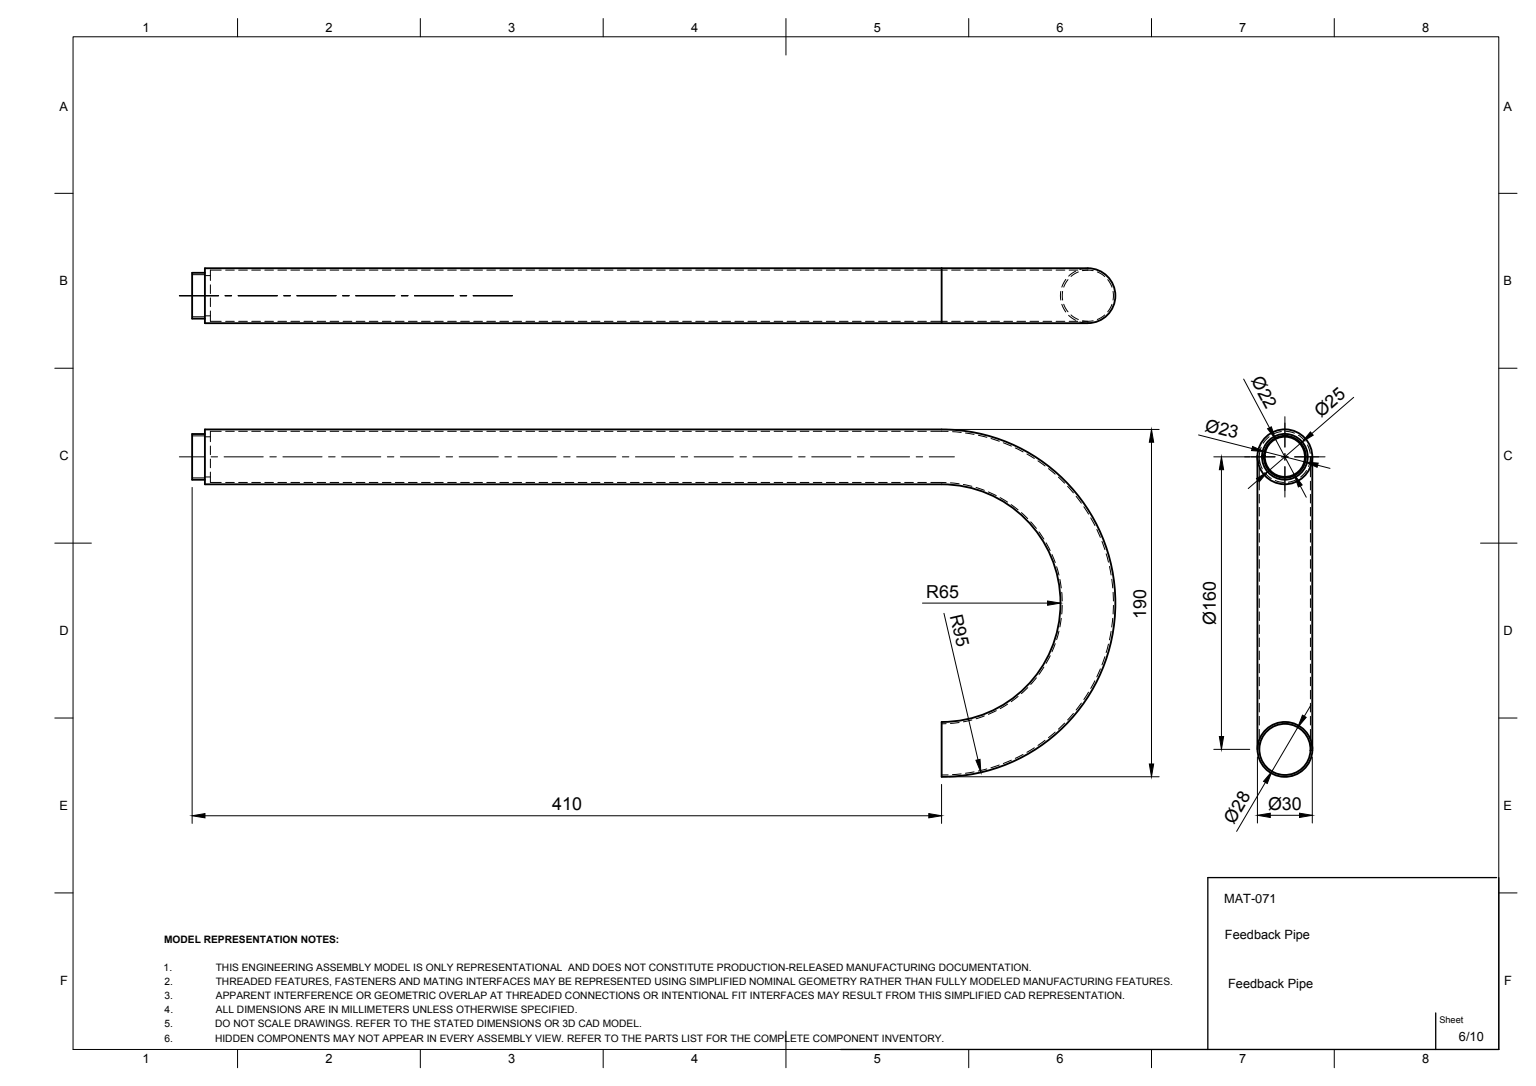
ISO-10303-21;
HEADER;
/* Generated by software containing ST-Developer
 * from STEP Tools, Inc. (www.steptools.com) 
 */

FILE_DESCRIPTION(
/* description */ (''),
/* implementation_level */ '2;1');

FILE_NAME(
/* name */ 'Feedback Pipe.step',
/* time_stamp */ '2026-10-24T12:24:47-07:00',
/* author */ (''),
/* organization */ (''),
/* preprocessor_version */ 'ST-DEVELOPER v20.2',
/* originating_system */ 'Autodesk Translation Framework v15.15.0.0',
/* authorisation */ '');

FILE_SCHEMA (('AUTOMOTIVE_DESIGN { 1 0 10303 214 3 1 1 }'));
ENDSEC;

DATA;
#10=MECHANICAL_DESIGN_GEOMETRIC_PRESENTATION_REPRESENTATION('',(#61),#13594);
#11=TOROIDAL_SURFACE('',#3227,80.0000000000001,15.);
#12=TOROIDAL_SURFACE('',#3233,80.0000000000001,14.);
#49=SHAPE_REPRESENTATION_RELATIONSHIP('SRR','None',#13629,#55);
#55=ADVANCED_BREP_SHAPE_REPRESENTATION('',(#67),#13592);
#61=STYLED_ITEM('',(#13667),#67);
#67=MANIFOLD_SOLID_BREP('Feedback Pipe',#2968);
#99=PLANE('',#3224);
#100=PLANE('',#3239);
#101=PLANE('',#3247);
#102=PLANE('',#3248);
#103=PLANE('',#3251);
#129=FACE_BOUND('',#538,.T.);
#130=FACE_BOUND('',#544,.T.);
#131=FACE_BOUND('',#548,.T.);
#132=FACE_BOUND('',#550,.T.);
#133=FACE_BOUND('',#553,.T.);
#185=CIRCLE('',#3225,15.);
#186=CIRCLE('',#3226,14.);
#187=CIRCLE('',#3228,15.);
#188=CIRCLE('',#3229,15.);
#189=CIRCLE('',#3230,65.0000000000001);
#190=CIRCLE('',#3232,15.);
#191=CIRCLE('',#3234,66.0000000000001);
#192=CIRCLE('',#3235,14.);
#193=CIRCLE('',#3236,14.);
#194=CIRCLE('',#3238,14.);
#195=CIRCLE('',#3240,11.);
#196=CIRCLE('',#3242,12.5);
#197=CIRCLE('',#3243,12.5);
#198=CIRCLE('',#3245,11.5);
#199=CIRCLE('',#3246,11.5);
#200=CIRCLE('',#3249,11.);
#350=FACE_OUTER_BOUND('',#537,.T.);
#351=FACE_OUTER_BOUND('',#539,.T.);
#352=FACE_OUTER_BOUND('',#540,.T.);
#353=FACE_OUTER_BOUND('',#541,.T.);
#354=FACE_OUTER_BOUND('',#542,.T.);
#355=FACE_OUTER_BOUND('',#543,.T.);
#356=FACE_OUTER_BOUND('',#545,.T.);
#357=FACE_OUTER_BOUND('',#546,.T.);
#358=FACE_OUTER_BOUND('',#547,.T.);
#359=FACE_OUTER_BOUND('',#549,.T.);
#360=FACE_OUTER_BOUND('',#551,.T.);
#361=FACE_OUTER_BOUND('',#552,.T.);
#537=EDGE_LOOP('',(#2555));
#538=EDGE_LOOP('',(#2556));
#539=EDGE_LOOP('',(#2557,#2558,#2559,#2560,#2561));
#540=EDGE_LOOP('',(#2562,#2563,#2564,#2565,#2566));
#541=EDGE_LOOP('',(#2567,#2568,#2569,#2570,#2571));
#542=EDGE_LOOP('',(#2572,#2573,#2574,#2575,#2576));
#543=EDGE_LOOP('',(#2577));
#544=EDGE_LOOP('',(#2578));
#545=EDGE_LOOP('',(#2579,#2580,#2581,#2582));
#546=EDGE_LOOP('',(#2583,#2584,#2585,#2586));
#547=EDGE_LOOP('',(#2587));
#548=EDGE_LOOP('',(#2588));
#549=EDGE_LOOP('',(#2589));
#550=EDGE_LOOP('',(#2590));
#551=EDGE_LOOP('',(#2591,#2592,#2593,#2594));
#552=EDGE_LOOP('',(#2595));
#553=EDGE_LOOP('',(#2596));
#908=LINE('',#11284,#1059);
#909=LINE('',#11293,#1060);
#910=LINE('',#11302,#1061);
#911=LINE('',#11308,#1062);
#912=LINE('',#11315,#1063);
#1059=VECTOR('',#3796,15.);
#1060=VECTOR('',#3807,14.);
#1061=VECTOR('',#3818,12.5);
#1062=VECTOR('',#3825,11.5);
#1063=VECTOR('',#3836,11.);
#1332=VERTEX_POINT('',#11271);
#1333=VERTEX_POINT('',#11273);
#1334=VERTEX_POINT('',#11276);
#1335=VERTEX_POINT('',#11277);
#1336=VERTEX_POINT('',#11282);
#1337=VERTEX_POINT('',#11286);
#1338=VERTEX_POINT('',#11288);
#1339=VERTEX_POINT('',#11292);
#1340=VERTEX_POINT('',#11296);
#1341=VERTEX_POINT('',#11299);
#1342=VERTEX_POINT('',#11301);
#1343=VERTEX_POINT('',#11305);
#1344=VERTEX_POINT('',#11307);
#1345=VERTEX_POINT('',#11312);
#1746=EDGE_CURVE('',#1332,#1332,#185,.T.);
#1747=EDGE_CURVE('',#1333,#1333,#186,.T.);
#1748=EDGE_CURVE('',#1334,#1335,#187,.T.);
#1749=EDGE_CURVE('',#1335,#1334,#188,.T.);
#1750=EDGE_CURVE('',#1334,#1332,#189,.T.);
#1751=EDGE_CURVE('',#1336,#1336,#190,.T.);
#1752=EDGE_CURVE('',#1336,#1335,#908,.T.);
#1753=EDGE_CURVE('',#1333,#1337,#191,.T.);
#1754=EDGE_CURVE('',#1338,#1337,#192,.T.);
#1755=EDGE_CURVE('',#1337,#1338,#193,.T.);
#1756=EDGE_CURVE('',#1338,#1339,#909,.T.);
#1757=EDGE_CURVE('',#1339,#1339,#194,.T.);
#1758=EDGE_CURVE('',#1340,#1340,#195,.T.);
#1759=EDGE_CURVE('',#1341,#1341,#196,.T.);
#1760=EDGE_CURVE('',#1341,#1342,#910,.T.);
#1761=EDGE_CURVE('',#1342,#1342,#197,.T.);
#1762=EDGE_CURVE('',#1343,#1343,#198,.T.);
#1763=EDGE_CURVE('',#1343,#1344,#911,.T.);
#1764=EDGE_CURVE('',#1344,#1344,#199,.T.);
#1765=EDGE_CURVE('',#1345,#1345,#200,.T.);
#1766=EDGE_CURVE('',#1345,#1340,#912,.T.);
#2555=ORIENTED_EDGE('',*,*,#1746,.T.);
#2556=ORIENTED_EDGE('',*,*,#1747,.F.);
#2557=ORIENTED_EDGE('',*,*,#1748,.T.);
#2558=ORIENTED_EDGE('',*,*,#1749,.T.);
#2559=ORIENTED_EDGE('',*,*,#1750,.T.);
#2560=ORIENTED_EDGE('',*,*,#1746,.F.);
#2561=ORIENTED_EDGE('',*,*,#1750,.F.);
#2562=ORIENTED_EDGE('',*,*,#1751,.T.);
#2563=ORIENTED_EDGE('',*,*,#1752,.T.);
#2564=ORIENTED_EDGE('',*,*,#1748,.F.);
#2565=ORIENTED_EDGE('',*,*,#1749,.F.);
#2566=ORIENTED_EDGE('',*,*,#1752,.F.);
#2567=ORIENTED_EDGE('',*,*,#1747,.T.);
#2568=ORIENTED_EDGE('',*,*,#1753,.T.);
#2569=ORIENTED_EDGE('',*,*,#1754,.F.);
#2570=ORIENTED_EDGE('',*,*,#1755,.F.);
#2571=ORIENTED_EDGE('',*,*,#1753,.F.);
#2572=ORIENTED_EDGE('',*,*,#1754,.T.);
#2573=ORIENTED_EDGE('',*,*,#1755,.T.);
#2574=ORIENTED_EDGE('',*,*,#1756,.T.);
#2575=ORIENTED_EDGE('',*,*,#1757,.F.);
#2576=ORIENTED_EDGE('',*,*,#1756,.F.);
#2577=ORIENTED_EDGE('',*,*,#1757,.T.);
#2578=ORIENTED_EDGE('',*,*,#1758,.F.);
#2579=ORIENTED_EDGE('',*,*,#1759,.T.);
#2580=ORIENTED_EDGE('',*,*,#1760,.T.);
#2581=ORIENTED_EDGE('',*,*,#1761,.F.);
#2582=ORIENTED_EDGE('',*,*,#1760,.F.);
#2583=ORIENTED_EDGE('',*,*,#1762,.T.);
#2584=ORIENTED_EDGE('',*,*,#1763,.T.);
#2585=ORIENTED_EDGE('',*,*,#1764,.F.);
#2586=ORIENTED_EDGE('',*,*,#1763,.F.);
#2587=ORIENTED_EDGE('',*,*,#1759,.F.);
#2588=ORIENTED_EDGE('',*,*,#1764,.T.);
#2589=ORIENTED_EDGE('',*,*,#1762,.F.);
#2590=ORIENTED_EDGE('',*,*,#1765,.T.);
#2591=ORIENTED_EDGE('',*,*,#1765,.F.);
#2592=ORIENTED_EDGE('',*,*,#1766,.T.);
#2593=ORIENTED_EDGE('',*,*,#1758,.T.);
#2594=ORIENTED_EDGE('',*,*,#1766,.F.);
#2595=ORIENTED_EDGE('',*,*,#1751,.F.);
#2596=ORIENTED_EDGE('',*,*,#1761,.T.);
#2785=CYLINDRICAL_SURFACE('',#3231,15.);
#2786=CYLINDRICAL_SURFACE('',#3237,14.);
#2787=CYLINDRICAL_SURFACE('',#3241,12.5);
#2788=CYLINDRICAL_SURFACE('',#3244,11.5);
#2789=CYLINDRICAL_SURFACE('',#3250,11.);
#2937=ADVANCED_FACE('',(#350,#129),#99,.T.);
#2938=ADVANCED_FACE('',(#351),#11,.T.);
#2939=ADVANCED_FACE('',(#352),#2785,.T.);
#2940=ADVANCED_FACE('',(#353),#12,.F.);
#2941=ADVANCED_FACE('',(#354),#2786,.F.);
#2942=ADVANCED_FACE('',(#355,#130),#100,.T.);
#2943=ADVANCED_FACE('',(#356),#2787,.T.);
#2944=ADVANCED_FACE('',(#357),#2788,.F.);
#2945=ADVANCED_FACE('',(#358,#131),#101,.F.);
#2946=ADVANCED_FACE('',(#359,#132),#102,.F.);
#2947=ADVANCED_FACE('',(#360),#2789,.F.);
#2948=ADVANCED_FACE('',(#361,#133),#103,.F.);
#2968=CLOSED_SHELL('',(#2937,#2938,#2939,#2940,#2941,#2942,#2943,#2944,
#2945,#2946,#2947,#2948));
#3223=AXIS2_PLACEMENT_3D('',#11269,#3776,#3777);
#3224=AXIS2_PLACEMENT_3D('',#11270,#3778,#3779);
#3225=AXIS2_PLACEMENT_3D('',#11272,#3780,#3781);
#3226=AXIS2_PLACEMENT_3D('',#11274,#3782,#3783);
#3227=AXIS2_PLACEMENT_3D('',#11275,#3784,#3785);
#3228=AXIS2_PLACEMENT_3D('',#11278,#3786,#3787);
#3229=AXIS2_PLACEMENT_3D('',#11279,#3788,#3789);
#3230=AXIS2_PLACEMENT_3D('',#11280,#3790,#3791);
#3231=AXIS2_PLACEMENT_3D('',#11281,#3792,#3793);
#3232=AXIS2_PLACEMENT_3D('',#11283,#3794,#3795);
#3233=AXIS2_PLACEMENT_3D('',#11285,#3797,#3798);
#3234=AXIS2_PLACEMENT_3D('',#11287,#3799,#3800);
#3235=AXIS2_PLACEMENT_3D('',#11289,#3801,#3802);
#3236=AXIS2_PLACEMENT_3D('',#11290,#3803,#3804);
#3237=AXIS2_PLACEMENT_3D('',#11291,#3805,#3806);
#3238=AXIS2_PLACEMENT_3D('',#11294,#3808,#3809);
#3239=AXIS2_PLACEMENT_3D('',#11295,#3810,#3811);
#3240=AXIS2_PLACEMENT_3D('',#11297,#3812,#3813);
#3241=AXIS2_PLACEMENT_3D('',#11298,#3814,#3815);
#3242=AXIS2_PLACEMENT_3D('',#11300,#3816,#3817);
#3243=AXIS2_PLACEMENT_3D('',#11303,#3819,#3820);
#3244=AXIS2_PLACEMENT_3D('',#11304,#3821,#3822);
#3245=AXIS2_PLACEMENT_3D('',#11306,#3823,#3824);
#3246=AXIS2_PLACEMENT_3D('',#11309,#3826,#3827);
#3247=AXIS2_PLACEMENT_3D('',#11310,#3828,#3829);
#3248=AXIS2_PLACEMENT_3D('',#11311,#3830,#3831);
#3249=AXIS2_PLACEMENT_3D('',#11313,#3832,#3833);
#3250=AXIS2_PLACEMENT_3D('',#11314,#3834,#3835);
#3251=AXIS2_PLACEMENT_3D('',#11316,#3837,#3838);
#3776=DIRECTION('axis',(0.,0.,1.));
#3777=DIRECTION('refdir',(1.,0.,0.));
#3778=DIRECTION('center_axis',(1.73472347597681E-16,-1.,-5.55111512312578E-16));
#3779=DIRECTION('ref_axis',(0.,5.55111512312578E-16,-1.));
#3780=DIRECTION('center_axis',(1.73472347597681E-16,-1.,-5.55111512312578E-16));
#3781=DIRECTION('ref_axis',(-1.,-1.73472347597681E-16,-9.62964972193618E-32));
#3782=DIRECTION('center_axis',(1.73472347597681E-16,-1.,-5.55111512312578E-16));
#3783=DIRECTION('ref_axis',(0.,5.55111512312578E-16,-1.));
#3784=DIRECTION('center_axis',(1.,0.,0.));
#3785=DIRECTION('ref_axis',(0.,0.,-1.));
#3786=DIRECTION('center_axis',(1.73472347597681E-16,1.,0.));
#3787=DIRECTION('ref_axis',(-1.,1.73472347597681E-16,0.));
#3788=DIRECTION('center_axis',(1.73472347597681E-16,1.,0.));
#3789=DIRECTION('ref_axis',(-1.,1.73472347597681E-16,0.));
#3790=DIRECTION('center_axis',(-1.,0.,0.));
#3791=DIRECTION('ref_axis',(0.,0.,-1.));
#3792=DIRECTION('center_axis',(0.,-1.,-1.38777878078145E-16));
#3793=DIRECTION('ref_axis',(0.,1.38777878078145E-16,-1.));
#3794=DIRECTION('center_axis',(1.73472347597681E-16,1.,0.));
#3795=DIRECTION('ref_axis',(-1.,1.73472347597681E-16,0.));
#3796=DIRECTION('',(0.,1.,1.38777878078145E-16));
#3797=DIRECTION('center_axis',(1.,0.,0.));
#3798=DIRECTION('ref_axis',(0.,0.,-1.));
#3799=DIRECTION('center_axis',(1.,0.,0.));
#3800=DIRECTION('ref_axis',(0.,0.,-1.));
#3801=DIRECTION('center_axis',(0.,1.,3.43024899888577E-15));
#3802=DIRECTION('ref_axis',(0.,-3.43024899888577E-15,1.));
#3803=DIRECTION('center_axis',(0.,1.,3.43024899888577E-15));
#3804=DIRECTION('ref_axis',(0.,-3.43024899888577E-15,1.));
#3805=DIRECTION('center_axis',(0.,-1.,-1.38777878078145E-16));
#3806=DIRECTION('ref_axis',(0.,1.38777878078145E-16,-1.));
#3807=DIRECTION('',(0.,-1.,-1.38777878078145E-16));
#3808=DIRECTION('center_axis',(1.73472347597681E-16,1.,0.));
#3809=DIRECTION('ref_axis',(-1.,1.73472347597681E-16,0.));
#3810=DIRECTION('center_axis',(1.73472347597681E-16,1.,0.));
#3811=DIRECTION('ref_axis',(0.,0.,1.));
#3812=DIRECTION('center_axis',(1.73472347597681E-16,1.,0.));
#3813=DIRECTION('ref_axis',(1.,-1.73472347597681E-16,0.));
#3814=DIRECTION('center_axis',(-1.73472347597681E-16,-1.,0.));
#3815=DIRECTION('ref_axis',(1.,-1.73472347597681E-16,0.));
#3816=DIRECTION('center_axis',(1.73472347597681E-16,1.,0.));
#3817=DIRECTION('ref_axis',(-1.,1.73472347597681E-16,0.));
#3818=DIRECTION('',(1.73472347597681E-16,1.,0.));
#3819=DIRECTION('center_axis',(1.73472347597681E-16,1.,0.));
#3820=DIRECTION('ref_axis',(-1.,1.73472347597681E-16,0.));
#3821=DIRECTION('center_axis',(-1.73472347597681E-16,-1.,0.));
#3822=DIRECTION('ref_axis',(1.,-1.73472347597681E-16,0.));
#3823=DIRECTION('center_axis',(1.73472347597681E-16,1.,0.));
#3824=DIRECTION('ref_axis',(-1.,1.73472347597681E-16,0.));
#3825=DIRECTION('',(-1.73472347597681E-16,-1.,0.));
#3826=DIRECTION('center_axis',(1.73472347597681E-16,1.,0.));
#3827=DIRECTION('ref_axis',(1.,-1.73472347597681E-16,0.));
#3828=DIRECTION('center_axis',(1.73472347597681E-16,1.,0.));
#3829=DIRECTION('ref_axis',(0.,0.,1.));
#3830=DIRECTION('center_axis',(1.73472347597681E-16,1.,0.));
#3831=DIRECTION('ref_axis',(0.,0.,1.));
#3832=DIRECTION('center_axis',(1.73472347597681E-16,1.,0.));
#3833=DIRECTION('ref_axis',(1.,-1.73472347597681E-16,0.));
#3834=DIRECTION('center_axis',(1.73472347597681E-16,1.,0.));
#3835=DIRECTION('ref_axis',(-1.,1.73472347597681E-16,0.));
#3836=DIRECTION('',(1.73472347597681E-16,1.,0.));
#3837=DIRECTION('center_axis',(1.73472347597681E-16,1.,0.));
#3838=DIRECTION('ref_axis',(0.,0.,1.));
#11269=CARTESIAN_POINT('',(0.,0.,0.));
#11270=CARTESIAN_POINT('Origin',(4.28614810332657E-14,460.,100.5));
#11271=CARTESIAN_POINT('',(4.10245108345447E-14,460.,115.5));
#11272=CARTESIAN_POINT('Origin',(4.28614810332657E-14,460.,100.5));
#11273=CARTESIAN_POINT('',(4.11469755144594E-14,460.,114.5));
#11274=CARTESIAN_POINT('Origin',(4.28614810332657E-14,460.,100.5));
#11275=CARTESIAN_POINT('Origin',(4.28614810332657E-14,460.,180.5));
#11276=CARTESIAN_POINT('',(4.10245108345447E-14,460.,245.5));
#11277=CARTESIAN_POINT('',(4.10245108345447E-14,460.,275.5));
#11278=CARTESIAN_POINT('Origin',(4.28614810332657E-14,460.,260.5));
#11279=CARTESIAN_POINT('Origin',(4.28614810332657E-14,460.,260.5));
#11280=CARTESIAN_POINT('Origin',(4.10245108345447E-14,460.,180.5));
#11281=CARTESIAN_POINT('Origin',(4.28614810332657E-14,460.,260.5));
#11282=CARTESIAN_POINT('',(4.10245108345447E-14,57.,275.5));
#11283=CARTESIAN_POINT('Origin',(4.23410639904727E-14,57.,260.5));
#11284=CARTESIAN_POINT('',(4.10245108345447E-14,460.,275.5));
#11285=CARTESIAN_POINT('Origin',(4.28614810332657E-14,460.,180.5));
#11286=CARTESIAN_POINT('',(4.11469755144594E-14,460.,246.5));
#11287=CARTESIAN_POINT('Origin',(4.11469755144594E-14,460.,180.5));
#11288=CARTESIAN_POINT('',(4.28614810332657E-14,460.,274.5));
#11289=CARTESIAN_POINT('Origin',(4.28614810332657E-14,460.,260.5));
#11290=CARTESIAN_POINT('Origin',(4.28614810332657E-14,460.,260.5));
#11291=CARTESIAN_POINT('Origin',(4.28614810332657E-14,460.,260.5));
#11292=CARTESIAN_POINT('',(4.11469755144594E-14,60.,274.5));
#11293=CARTESIAN_POINT('',(4.11469755144594E-14,460.,274.5));
#11294=CARTESIAN_POINT('Origin',(4.28614810332657E-14,60.,260.5));
#11295=CARTESIAN_POINT('Origin',(4.28614810332657E-14,60.,260.5));
#11296=CARTESIAN_POINT('',(11.,60.,260.5));
#11297=CARTESIAN_POINT('Origin',(4.28614810332657E-14,60.,260.5));
#11298=CARTESIAN_POINT('Origin',(4.28614810332657E-14,60.,260.5));
#11299=CARTESIAN_POINT('',(-12.5,50.,260.5));
#11300=CARTESIAN_POINT('Origin',(4.11267575572889E-14,50.,260.5));
#11301=CARTESIAN_POINT('',(-12.5,57.,260.5));
#11302=CARTESIAN_POINT('',(-12.5,60.,260.5));
#11303=CARTESIAN_POINT('Origin',(4.23410639904727E-14,57.,260.5));
#11304=CARTESIAN_POINT('Origin',(4.28614810332657E-14,60.,260.5));
#11305=CARTESIAN_POINT('',(-11.5,57.,260.5));
#11306=CARTESIAN_POINT('Origin',(4.23410639904727E-14,57.,260.5));
#11307=CARTESIAN_POINT('',(-11.5,50.,260.5));
#11308=CARTESIAN_POINT('',(-11.5,60.,260.5));
#11309=CARTESIAN_POINT('Origin',(4.11267575572889E-14,50.,260.5));
#11310=CARTESIAN_POINT('Origin',(4.11267575572889E-14,50.,260.5));
#11311=CARTESIAN_POINT('Origin',(4.23410639904727E-14,57.,260.5));
#11312=CARTESIAN_POINT('',(11.,57.,260.5));
#11313=CARTESIAN_POINT('Origin',(4.23410639904727E-14,57.,260.5));
#11314=CARTESIAN_POINT('Origin',(4.23410639904727E-14,57.,260.5));
#11315=CARTESIAN_POINT('',(11.,57.,260.5));
#11316=CARTESIAN_POINT('Origin',(4.23410639904727E-14,57.,260.5));
#13583=UNCERTAINTY_MEASURE_WITH_UNIT(LENGTH_MEASURE(0.01),#13595,
'DISTANCE_ACCURACY_VALUE',
'Maximum model space distance between geometric entities at asserted c
onnectivities');
#13585=UNCERTAINTY_MEASURE_WITH_UNIT(LENGTH_MEASURE(0.01),#13595,
'DISTANCE_ACCURACY_VALUE',
'Maximum model space distance between geometric entities at asserted c
onnectivities');
#13592=(
GEOMETRIC_REPRESENTATION_CONTEXT(3)
GLOBAL_UNCERTAINTY_ASSIGNED_CONTEXT((#13583))
GLOBAL_UNIT_ASSIGNED_CONTEXT((#13595,#13597,#13598))
REPRESENTATION_CONTEXT('','3D')
);
#13594=(
GEOMETRIC_REPRESENTATION_CONTEXT(3)
GLOBAL_UNCERTAINTY_ASSIGNED_CONTEXT((#13585))
GLOBAL_UNIT_ASSIGNED_CONTEXT((#13595,#13597,#13598))
REPRESENTATION_CONTEXT('','3D')
);
#13595=(
LENGTH_UNIT()
NAMED_UNIT(*)
SI_UNIT(.MILLI.,.METRE.)
);
#13597=(
NAMED_UNIT(*)
PLANE_ANGLE_UNIT()
SI_UNIT($,.RADIAN.)
);
#13598=(
NAMED_UNIT(*)
SI_UNIT($,.STERADIAN.)
SOLID_ANGLE_UNIT()
);
#13605=SHAPE_DEFINITION_REPRESENTATION(#13616,#13629);
#13616=PRODUCT_DEFINITION_SHAPE('',$,#13638);
#13629=SHAPE_REPRESENTATION('',(#3223),#13592);
#13631=PRODUCT_DEFINITION_CONTEXT('part definition',#13657,'design');
#13638=PRODUCT_DEFINITION('Feedback Pipe','Feedback Pipe',#13646,#13631);
#13646=PRODUCT_DEFINITION_FORMATION('',$,#13665);
#13657=APPLICATION_CONTEXT(
'Core Data for Automotive Mechanical Design Process');
#13658=PRODUCT_CONTEXT('part definition',#13657,'mechanical');
#13665=PRODUCT('Feedback Pipe','Feedback Pipe',$,(#13658));
#13667=PRESENTATION_STYLE_ASSIGNMENT((#13668));
#13668=SURFACE_STYLE_USAGE(.BOTH.,#13669);
#13669=SURFACE_SIDE_STYLE('',(#13670));
#13670=SURFACE_STYLE_FILL_AREA(#13671);
#13671=FILL_AREA_STYLE('Steel - Satin',(#13672));
#13672=FILL_AREA_STYLE_COLOUR('Steel - Satin',#13673);
#13673=COLOUR_RGB('Steel - Satin',0.627450980392157,0.627450980392157,0.627450980392157);
ENDSEC;
END-ISO-10303-21;
